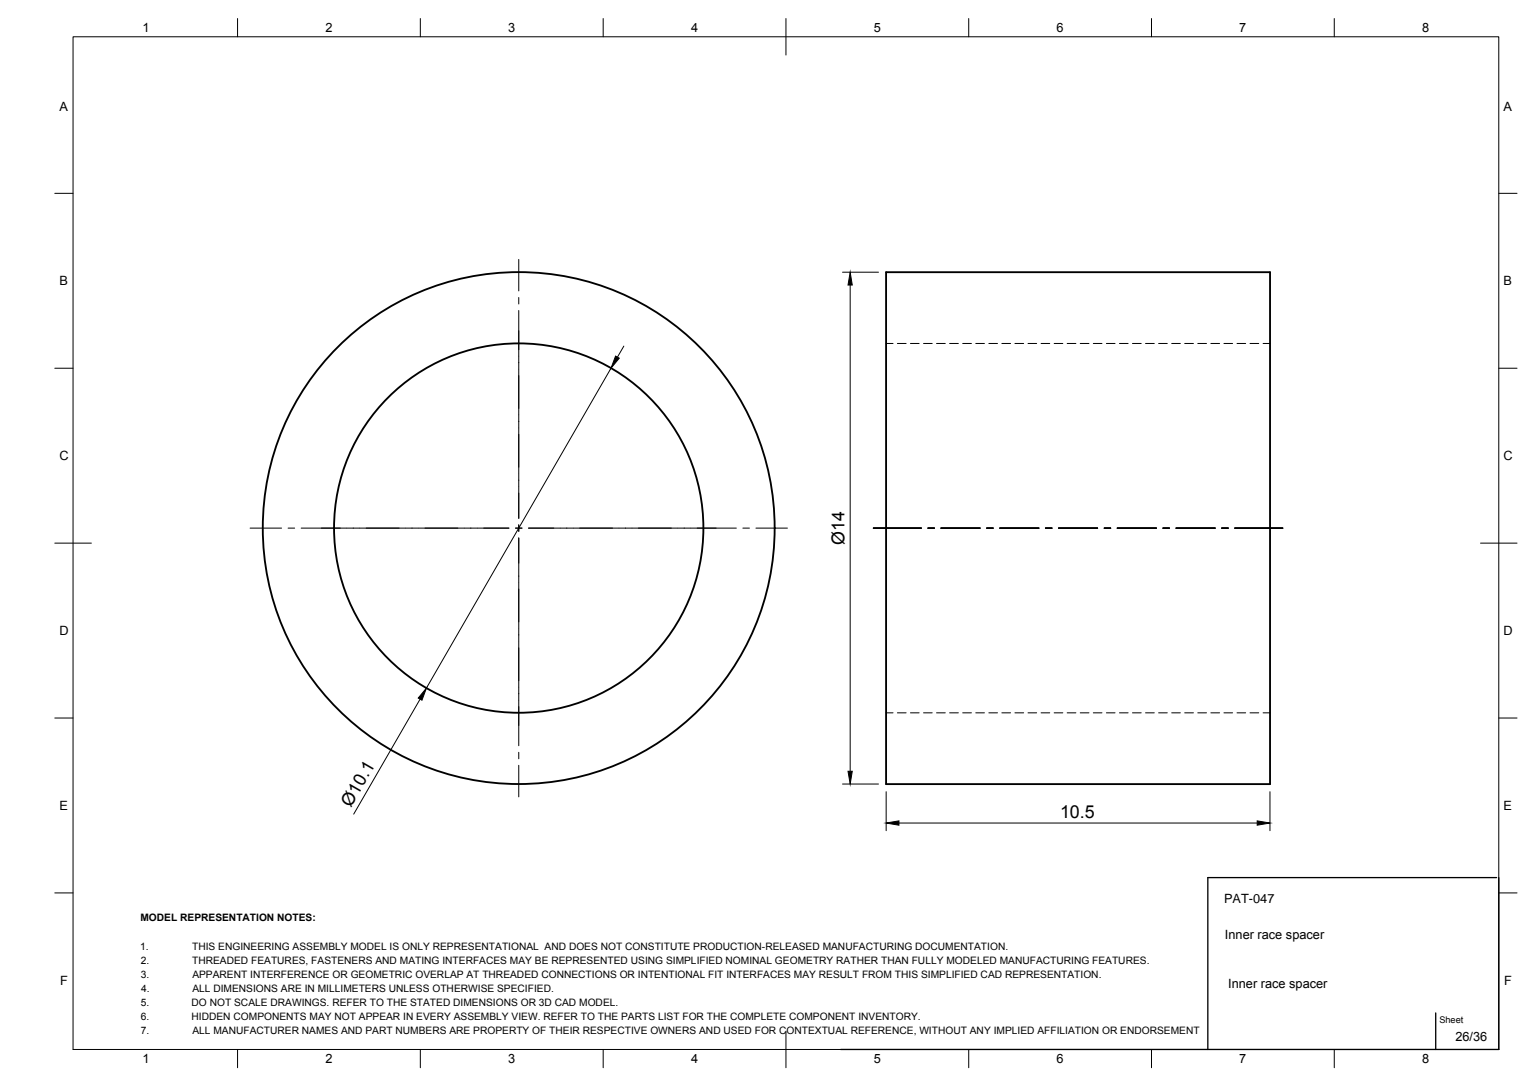
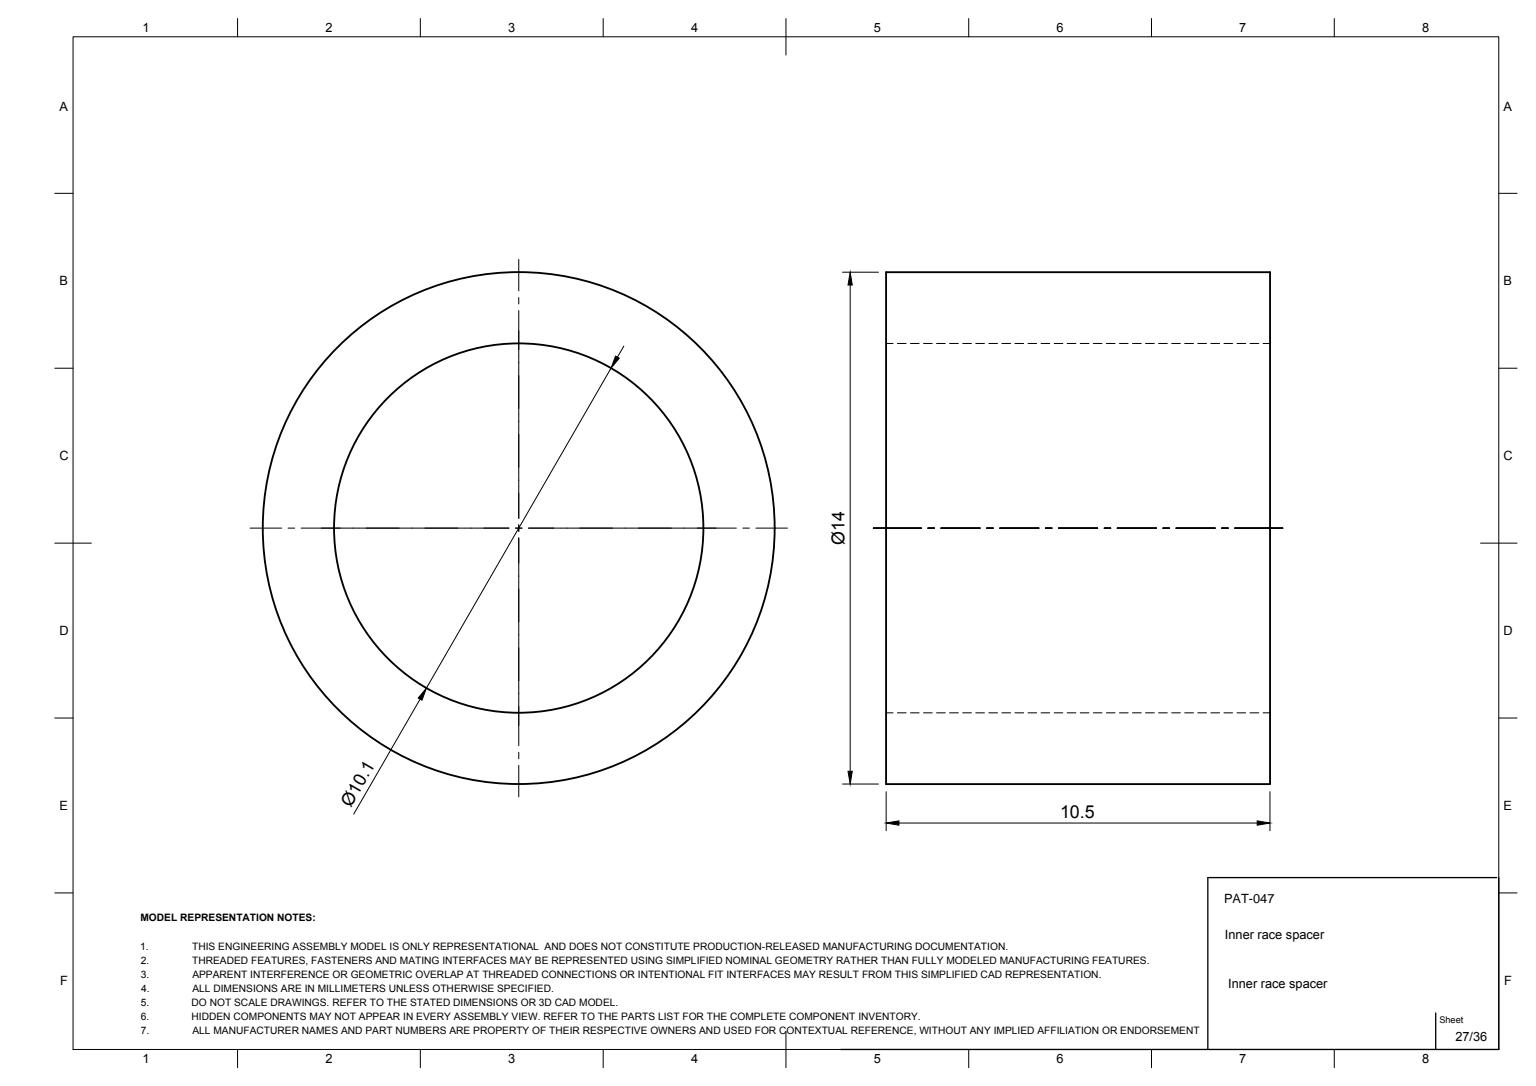
ISO-10303-21;
HEADER;
/* Generated by software containing ST-Developer
 * from STEP Tools, Inc. (www.steptools.com) 
 */

FILE_DESCRIPTION(
/* description */ ('Gravity roller conveyor section'),
/* implementation_level */ '2;1');

FILE_NAME(
/* name */ 'Inner race spacer.step',
/* time_stamp */ '2026-11-02T07:43:02-08:00',
/* author */ (''),
/* organization */ (''),
/* preprocessor_version */ 'ST-DEVELOPER v20.2',
/* originating_system */ 'Autodesk Translation Framework v15.17.0.0',
/* authorisation */ '');

FILE_SCHEMA (('AUTOMOTIVE_DESIGN { 1 0 10303 214 3 1 1 }'));
ENDSEC;

DATA;
#10=MECHANICAL_DESIGN_GEOMETRIC_PRESENTATION_REPRESENTATION('',(#551),#13821);
#483=SHAPE_REPRESENTATION_RELATIONSHIP('SRR','None',#14021,#517);
#517=ADVANCED_BREP_SHAPE_REPRESENTATION('',(#591),#13808);
#551=STYLED_ITEM('',(#14191),#591);
#591=MANIFOLD_SOLID_BREP('Body1',#7651);
#676=FACE_BOUND('',#1793,.T.);
#677=FACE_BOUND('',#1795,.T.);
#941=PLANE('',#8481);
#942=PLANE('',#8482);
#1304=FACE_OUTER_BOUND('',#1790,.T.);
#1305=FACE_OUTER_BOUND('',#1791,.T.);
#1306=FACE_OUTER_BOUND('',#1792,.T.);
#1307=FACE_OUTER_BOUND('',#1794,.T.);
#1790=EDGE_LOOP('',(#6630,#6631,#6632,#6633));
#1791=EDGE_LOOP('',(#6634,#6635,#6636,#6637));
#1792=EDGE_LOOP('',(#6638));
#1793=EDGE_LOOP('',(#6639));
#1794=EDGE_LOOP('',(#6640));
#1795=EDGE_LOOP('',(#6641));
#2538=LINE('',#12758,#3256);
#2539=LINE('',#12764,#3257);
#3256=VECTOR('',#10275,0.505);
#3257=VECTOR('',#10282,0.7);
#3478=CIRCLE('',#8476,0.505);
#3479=CIRCLE('',#8477,0.505);
#3480=CIRCLE('',#8479,0.7);
#3481=CIRCLE('',#8480,0.7);
#4064=VERTEX_POINT('',#12755);
#4065=VERTEX_POINT('',#12757);
#4066=VERTEX_POINT('',#12761);
#4067=VERTEX_POINT('',#12763);
#4952=EDGE_CURVE('',#4064,#4064,#3478,.T.);
#4953=EDGE_CURVE('',#4064,#4065,#2538,.T.);
#4954=EDGE_CURVE('',#4065,#4065,#3479,.T.);
#4955=EDGE_CURVE('',#4066,#4066,#3480,.T.);
#4956=EDGE_CURVE('',#4066,#4067,#2539,.T.);
#4957=EDGE_CURVE('',#4067,#4067,#3481,.T.);
#6630=ORIENTED_EDGE('',*,*,#4952,.F.);
#6631=ORIENTED_EDGE('',*,*,#4953,.T.);
#6632=ORIENTED_EDGE('',*,*,#4954,.T.);
#6633=ORIENTED_EDGE('',*,*,#4953,.F.);
#6634=ORIENTED_EDGE('',*,*,#4955,.F.);
#6635=ORIENTED_EDGE('',*,*,#4956,.T.);
#6636=ORIENTED_EDGE('',*,*,#4957,.T.);
#6637=ORIENTED_EDGE('',*,*,#4956,.F.);
#6638=ORIENTED_EDGE('',*,*,#4955,.T.);
#6639=ORIENTED_EDGE('',*,*,#4952,.T.);
#6640=ORIENTED_EDGE('',*,*,#4957,.F.);
#6641=ORIENTED_EDGE('',*,*,#4954,.F.);
#7180=CYLINDRICAL_SURFACE('',#8475,0.505);
#7181=CYLINDRICAL_SURFACE('',#8478,0.7);
#7505=ADVANCED_FACE('',(#1304),#7180,.F.);
#7506=ADVANCED_FACE('',(#1305),#7181,.T.);
#7507=ADVANCED_FACE('',(#1306,#676),#941,.T.);
#7508=ADVANCED_FACE('',(#1307,#677),#942,.F.);
#7651=CLOSED_SHELL('',(#7505,#7506,#7507,#7508));
#8474=AXIS2_PLACEMENT_3D('',#12753,#10269,#10270);
#8475=AXIS2_PLACEMENT_3D('',#12754,#10271,#10272);
#8476=AXIS2_PLACEMENT_3D('',#12756,#10273,#10274);
#8477=AXIS2_PLACEMENT_3D('',#12759,#10276,#10277);
#8478=AXIS2_PLACEMENT_3D('',#12760,#10278,#10279);
#8479=AXIS2_PLACEMENT_3D('',#12762,#10280,#10281);
#8480=AXIS2_PLACEMENT_3D('',#12765,#10283,#10284);
#8481=AXIS2_PLACEMENT_3D('',#12766,#10285,#10286);
#8482=AXIS2_PLACEMENT_3D('',#12767,#10287,#10288);
#10269=DIRECTION('axis',(0.,0.,1.));
#10270=DIRECTION('refdir',(1.,0.,0.));
#10271=DIRECTION('center_axis',(0.,1.,0.));
#10272=DIRECTION('ref_axis',(1.,0.,0.));
#10273=DIRECTION('center_axis',(0.,-1.,0.));
#10274=DIRECTION('ref_axis',(1.,0.,0.));
#10275=DIRECTION('',(0.,-1.,0.));
#10276=DIRECTION('center_axis',(0.,-1.,0.));
#10277=DIRECTION('ref_axis',(1.,0.,0.));
#10278=DIRECTION('center_axis',(0.,1.,0.));
#10279=DIRECTION('ref_axis',(1.,0.,0.));
#10280=DIRECTION('center_axis',(0.,1.,0.));
#10281=DIRECTION('ref_axis',(1.,0.,0.));
#10282=DIRECTION('',(0.,-1.,0.));
#10283=DIRECTION('center_axis',(0.,1.,0.));
#10284=DIRECTION('ref_axis',(1.,0.,0.));
#10285=DIRECTION('center_axis',(0.,1.,0.));
#10286=DIRECTION('ref_axis',(1.,0.,0.));
#10287=DIRECTION('center_axis',(0.,1.,0.));
#10288=DIRECTION('ref_axis',(1.,0.,0.));
#12753=CARTESIAN_POINT('',(0.,0.,0.));
#12754=CARTESIAN_POINT('Origin',(3.,-1.,8.));
#12755=CARTESIAN_POINT('',(2.495,0.05,8.));
#12756=CARTESIAN_POINT('Origin',(3.,0.05,8.));
#12757=CARTESIAN_POINT('',(2.495,-1.,8.));
#12758=CARTESIAN_POINT('',(2.495,-1.,8.));
#12759=CARTESIAN_POINT('Origin',(3.,-1.,8.));
#12760=CARTESIAN_POINT('Origin',(3.,-1.,8.));
#12761=CARTESIAN_POINT('',(2.3,0.05,8.));
#12762=CARTESIAN_POINT('Origin',(3.,0.05,8.));
#12763=CARTESIAN_POINT('',(2.3,-1.,8.));
#12764=CARTESIAN_POINT('',(2.3,-1.,8.));
#12765=CARTESIAN_POINT('Origin',(3.,-1.,8.));
#12766=CARTESIAN_POINT('Origin',(3.,0.05,8.));
#12767=CARTESIAN_POINT('Origin',(3.,-1.,8.));
#13769=UNCERTAINTY_MEASURE_WITH_UNIT(LENGTH_MEASURE(0.001),#13822,
'DISTANCE_ACCURACY_VALUE',
'Maximum model space distance between geometric entities at asserted c
onnectivities');
#13782=UNCERTAINTY_MEASURE_WITH_UNIT(LENGTH_MEASURE(0.001),#13822,
'DISTANCE_ACCURACY_VALUE',
'Maximum model space distance between geometric entities at asserted c
onnectivities');
#13808=(
GEOMETRIC_REPRESENTATION_CONTEXT(3)
GLOBAL_UNCERTAINTY_ASSIGNED_CONTEXT((#13769))
GLOBAL_UNIT_ASSIGNED_CONTEXT((#13822,#13824,#13825))
REPRESENTATION_CONTEXT('','3D')
);
#13821=(
GEOMETRIC_REPRESENTATION_CONTEXT(3)
GLOBAL_UNCERTAINTY_ASSIGNED_CONTEXT((#13782))
GLOBAL_UNIT_ASSIGNED_CONTEXT((#13822,#13824,#13825))
REPRESENTATION_CONTEXT('','3D')
);
#13822=(
LENGTH_UNIT()
NAMED_UNIT(*)
SI_UNIT(.CENTI.,.METRE.)
);
#13824=(
NAMED_UNIT(*)
PLANE_ANGLE_UNIT()
SI_UNIT($,.RADIAN.)
);
#13825=(
NAMED_UNIT(*)
SI_UNIT($,.STERADIAN.)
SOLID_ANGLE_UNIT()
);
#13851=SHAPE_DEFINITION_REPRESENTATION(#13889,#14021);
#13889=PRODUCT_DEFINITION_SHAPE('',$,#14060);
#14021=SHAPE_REPRESENTATION('',(#8474),#13808);
#14034=PRODUCT_DEFINITION_CONTEXT('part definition',#14150,'design');
#14060=PRODUCT_DEFINITION('Inner race spacer','Inner race spacer',#14098,
#14034);
#14098=PRODUCT_DEFINITION_FORMATION('',$,#14177);
#14150=APPLICATION_CONTEXT(
'Core Data for Automotive Mechanical Design Process');
#14151=PRODUCT_CONTEXT('part definition',#14150,'mechanical');
#14177=PRODUCT('Inner race spacer','Inner race spacer',
'Inner race spacer',(#14151));
#14191=PRESENTATION_STYLE_ASSIGNMENT((#14196));
#14196=SURFACE_STYLE_USAGE(.BOTH.,#14201);
#14201=SURFACE_SIDE_STYLE('',(#14206));
#14206=SURFACE_STYLE_FILL_AREA(#14211);
#14211=FILL_AREA_STYLE('CAD Library Painted - Steel gray',(#14216));
#14216=FILL_AREA_STYLE_COLOUR('CAD Library Painted - Steel gray',#14221);
#14221=COLOUR_RGB('CAD Library Painted - Steel gray',0.592156862745098,
0.631372549019608,0.67843137254902);
ENDSEC;
END-ISO-10303-21;
